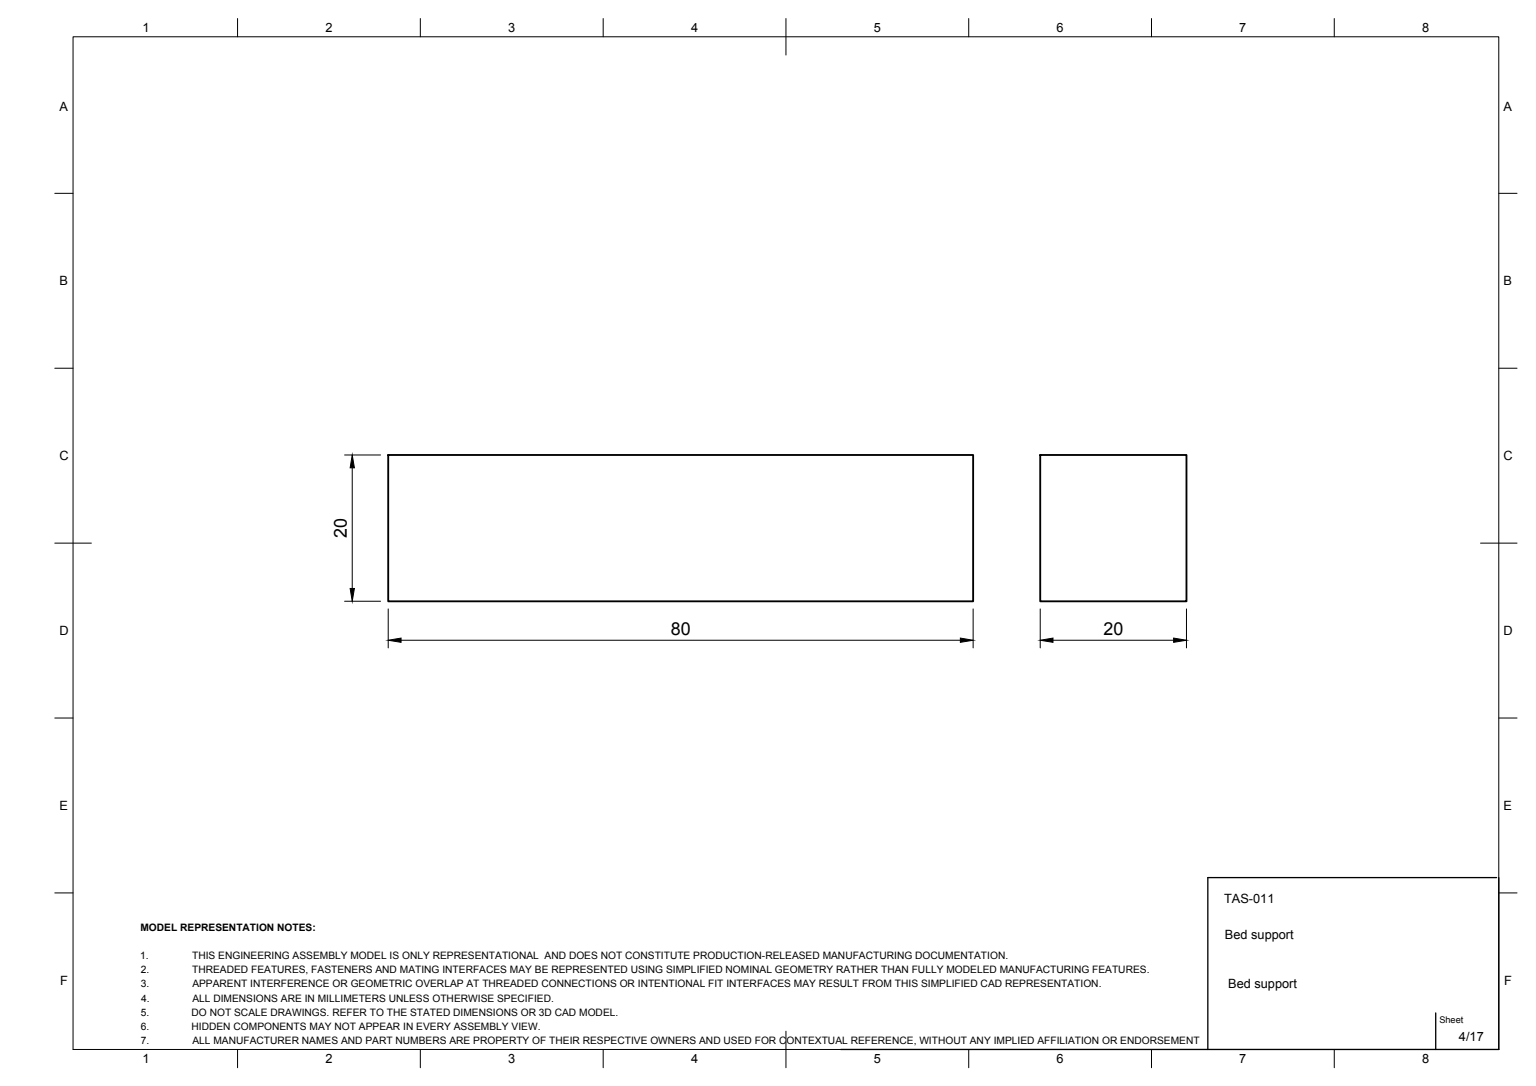
ISO-10303-21;
HEADER;
/* Generated by software containing ST-Developer
 * from STEP Tools, Inc. (www.steptools.com) 
 */

FILE_DESCRIPTION(
/* description */ (
'Independent manual bench leaf bending machine,200mm work width. Fabri
cated welded frame and folding leaf, repeated bushed and fully retaine
d hinge hardware, two handles with bonded grips, beveled clamping beam
 and modeledM12 clamp screws.2mm omitted-workpiece assembly reference 
gap, not a capacity claim. Native135deg hinge travel. Weld sizing, pro
duction fits, material condition, bending capacity, strength and life 
unassigned.'),
/* implementation_level */ '2;1');

FILE_NAME(
/* name */ 'Bed support.step',
/* time_stamp */ '2026-11-14T09:11:34-08:00',
/* author */ (''),
/* organization */ (''),
/* preprocessor_version */ 'ST-DEVELOPER v20.2',
/* originating_system */ 'Autodesk Translation Framework v15.17.0.0',
/* authorisation */ '');

FILE_SCHEMA (('AUTOMOTIVE_DESIGN { 1 0 10303 214 3 1 1 }'));
ENDSEC;

DATA;
#10=MECHANICAL_DESIGN_GEOMETRIC_PRESENTATION_REPRESENTATION('',(#450),#37701);
#414=SHAPE_REPRESENTATION_RELATIONSHIP('SRR','None',#37783,#432);
#432=ADVANCED_BREP_SHAPE_REPRESENTATION('',(#468),#37687);
#450=STYLED_ITEM('',(#37882),#468);
#468=MANIFOLD_SOLID_BREP('Body1',#4148);
#540=PLANE('',#4435);
#541=PLANE('',#4436);
#542=PLANE('',#4437);
#543=PLANE('',#4438);
#544=PLANE('',#4439);
#545=PLANE('',#4440);
#642=FACE_OUTER_BOUND('',#870,.T.);
#643=FACE_OUTER_BOUND('',#871,.T.);
#644=FACE_OUTER_BOUND('',#872,.T.);
#645=FACE_OUTER_BOUND('',#873,.T.);
#646=FACE_OUTER_BOUND('',#874,.T.);
#647=FACE_OUTER_BOUND('',#875,.T.);
#870=EDGE_LOOP('',(#2823,#2824,#2825,#2826));
#871=EDGE_LOOP('',(#2827,#2828,#2829,#2830));
#872=EDGE_LOOP('',(#2831,#2832,#2833,#2834));
#873=EDGE_LOOP('',(#2835,#2836,#2837,#2838));
#874=EDGE_LOOP('',(#2839,#2840,#2841,#2842));
#875=EDGE_LOOP('',(#2843,#2844,#2845,#2846));
#1124=LINE('',#5849,#1373);
#1125=LINE('',#5851,#1374);
#1126=LINE('',#5853,#1375);
#1127=LINE('',#5854,#1376);
#1128=LINE('',#5857,#1377);
#1129=LINE('',#5859,#1378);
#1130=LINE('',#5860,#1379);
#1131=LINE('',#5863,#1380);
#1132=LINE('',#5865,#1381);
#1133=LINE('',#5866,#1382);
#1134=LINE('',#5868,#1383);
#1135=LINE('',#5869,#1384);
#1373=VECTOR('',#4921,10.);
#1374=VECTOR('',#4922,10.);
#1375=VECTOR('',#4923,10.);
#1376=VECTOR('',#4924,10.);
#1377=VECTOR('',#4927,10.);
#1378=VECTOR('',#4928,10.);
#1379=VECTOR('',#4929,10.);
#1380=VECTOR('',#4932,10.);
#1381=VECTOR('',#4933,10.);
#1382=VECTOR('',#4934,10.);
#1383=VECTOR('',#4937,10.);
#1384=VECTOR('',#4938,10.);
#1697=VERTEX_POINT('',#5847);
#1698=VERTEX_POINT('',#5848);
#1699=VERTEX_POINT('',#5850);
#1700=VERTEX_POINT('',#5852);
#1701=VERTEX_POINT('',#5856);
#1702=VERTEX_POINT('',#5858);
#1703=VERTEX_POINT('',#5862);
#1704=VERTEX_POINT('',#5864);
#2145=EDGE_CURVE('',#1697,#1698,#1124,.T.);
#2146=EDGE_CURVE('',#1698,#1699,#1125,.T.);
#2147=EDGE_CURVE('',#1700,#1699,#1126,.T.);
#2148=EDGE_CURVE('',#1697,#1700,#1127,.T.);
#2149=EDGE_CURVE('',#1701,#1697,#1128,.T.);
#2150=EDGE_CURVE('',#1702,#1700,#1129,.T.);
#2151=EDGE_CURVE('',#1701,#1702,#1130,.T.);
#2152=EDGE_CURVE('',#1703,#1701,#1131,.T.);
#2153=EDGE_CURVE('',#1704,#1702,#1132,.T.);
#2154=EDGE_CURVE('',#1703,#1704,#1133,.T.);
#2155=EDGE_CURVE('',#1698,#1703,#1134,.T.);
#2156=EDGE_CURVE('',#1699,#1704,#1135,.T.);
#2823=ORIENTED_EDGE('',*,*,#2145,.T.);
#2824=ORIENTED_EDGE('',*,*,#2146,.T.);
#2825=ORIENTED_EDGE('',*,*,#2147,.F.);
#2826=ORIENTED_EDGE('',*,*,#2148,.F.);
#2827=ORIENTED_EDGE('',*,*,#2149,.T.);
#2828=ORIENTED_EDGE('',*,*,#2148,.T.);
#2829=ORIENTED_EDGE('',*,*,#2150,.F.);
#2830=ORIENTED_EDGE('',*,*,#2151,.F.);
#2831=ORIENTED_EDGE('',*,*,#2152,.T.);
#2832=ORIENTED_EDGE('',*,*,#2151,.T.);
#2833=ORIENTED_EDGE('',*,*,#2153,.F.);
#2834=ORIENTED_EDGE('',*,*,#2154,.F.);
#2835=ORIENTED_EDGE('',*,*,#2155,.T.);
#2836=ORIENTED_EDGE('',*,*,#2154,.T.);
#2837=ORIENTED_EDGE('',*,*,#2156,.F.);
#2838=ORIENTED_EDGE('',*,*,#2146,.F.);
#2839=ORIENTED_EDGE('',*,*,#2156,.T.);
#2840=ORIENTED_EDGE('',*,*,#2153,.T.);
#2841=ORIENTED_EDGE('',*,*,#2150,.T.);
#2842=ORIENTED_EDGE('',*,*,#2147,.T.);
#2843=ORIENTED_EDGE('',*,*,#2155,.F.);
#2844=ORIENTED_EDGE('',*,*,#2145,.F.);
#2845=ORIENTED_EDGE('',*,*,#2149,.F.);
#2846=ORIENTED_EDGE('',*,*,#2152,.F.);
#3972=ADVANCED_FACE('',(#642),#540,.T.);
#3973=ADVANCED_FACE('',(#643),#541,.T.);
#3974=ADVANCED_FACE('',(#644),#542,.T.);
#3975=ADVANCED_FACE('',(#645),#543,.T.);
#3976=ADVANCED_FACE('',(#646),#544,.T.);
#3977=ADVANCED_FACE('',(#647),#545,.F.);
#4148=CLOSED_SHELL('',(#3972,#3973,#3974,#3975,#3976,#3977));
#4434=AXIS2_PLACEMENT_3D('',#5845,#4917,#4918);
#4435=AXIS2_PLACEMENT_3D('',#5846,#4919,#4920);
#4436=AXIS2_PLACEMENT_3D('',#5855,#4925,#4926);
#4437=AXIS2_PLACEMENT_3D('',#5861,#4930,#4931);
#4438=AXIS2_PLACEMENT_3D('',#5867,#4935,#4936);
#4439=AXIS2_PLACEMENT_3D('',#5870,#4939,#4940);
#4440=AXIS2_PLACEMENT_3D('',#5871,#4941,#4942);
#4917=DIRECTION('axis',(0.,0.,1.));
#4918=DIRECTION('refdir',(1.,0.,0.));
#4919=DIRECTION('center_axis',(0.,1.,0.));
#4920=DIRECTION('ref_axis',(-1.,0.,0.));
#4921=DIRECTION('',(-1.,0.,0.));
#4922=DIRECTION('',(0.,0.,1.));
#4923=DIRECTION('',(-1.,0.,0.));
#4924=DIRECTION('',(0.,0.,1.));
#4925=DIRECTION('center_axis',(1.,0.,0.));
#4926=DIRECTION('ref_axis',(0.,1.,0.));
#4927=DIRECTION('',(0.,1.,0.));
#4928=DIRECTION('',(0.,1.,0.));
#4929=DIRECTION('',(0.,0.,1.));
#4930=DIRECTION('center_axis',(0.,-1.,0.));
#4931=DIRECTION('ref_axis',(1.,0.,0.));
#4932=DIRECTION('',(1.,0.,0.));
#4933=DIRECTION('',(1.,0.,0.));
#4934=DIRECTION('',(0.,0.,1.));
#4935=DIRECTION('center_axis',(-1.,0.,0.));
#4936=DIRECTION('ref_axis',(0.,-1.,0.));
#4937=DIRECTION('',(0.,-1.,0.));
#4938=DIRECTION('',(0.,-1.,0.));
#4939=DIRECTION('center_axis',(0.,0.,1.));
#4940=DIRECTION('ref_axis',(1.,0.,0.));
#4941=DIRECTION('center_axis',(0.,0.,1.));
#4942=DIRECTION('ref_axis',(1.,0.,0.));
#5845=CARTESIAN_POINT('',(0.,0.,0.));
#5846=CARTESIAN_POINT('Origin',(-10.,10.,10.));
#5847=CARTESIAN_POINT('',(-10.,10.,10.));
#5848=CARTESIAN_POINT('',(-90.,10.,10.));
#5849=CARTESIAN_POINT('',(-10.,10.,10.));
#5850=CARTESIAN_POINT('',(-90.,10.,30.));
#5851=CARTESIAN_POINT('',(-90.,10.,10.));
#5852=CARTESIAN_POINT('',(-10.,10.,30.));
#5853=CARTESIAN_POINT('',(-10.,10.,30.));
#5854=CARTESIAN_POINT('',(-10.,10.,10.));
#5855=CARTESIAN_POINT('Origin',(-10.,-10.,10.));
#5856=CARTESIAN_POINT('',(-10.,-10.,10.));
#5857=CARTESIAN_POINT('',(-10.,-10.,10.));
#5858=CARTESIAN_POINT('',(-10.,-10.,30.));
#5859=CARTESIAN_POINT('',(-10.,-10.,30.));
#5860=CARTESIAN_POINT('',(-10.,-10.,10.));
#5861=CARTESIAN_POINT('Origin',(-90.,-10.,10.));
#5862=CARTESIAN_POINT('',(-90.,-10.,10.));
#5863=CARTESIAN_POINT('',(-90.,-10.,10.));
#5864=CARTESIAN_POINT('',(-90.,-10.,30.));
#5865=CARTESIAN_POINT('',(-90.,-10.,30.));
#5866=CARTESIAN_POINT('',(-90.,-10.,10.));
#5867=CARTESIAN_POINT('Origin',(-90.,10.,10.));
#5868=CARTESIAN_POINT('',(-90.,10.,10.));
#5869=CARTESIAN_POINT('',(-90.,10.,30.));
#5870=CARTESIAN_POINT('Origin',(-50.,0.,30.));
#5871=CARTESIAN_POINT('Origin',(-50.,0.,10.));
#37667=UNCERTAINTY_MEASURE_WITH_UNIT(LENGTH_MEASURE(0.01),#37702,
'DISTANCE_ACCURACY_VALUE',
'Maximum model space distance between geometric entities at asserted c
onnectivities');
#37681=UNCERTAINTY_MEASURE_WITH_UNIT(LENGTH_MEASURE(0.01),#37702,
'DISTANCE_ACCURACY_VALUE',
'Maximum model space distance between geometric entities at asserted c
onnectivities');
#37687=(
GEOMETRIC_REPRESENTATION_CONTEXT(3)
GLOBAL_UNCERTAINTY_ASSIGNED_CONTEXT((#37667))
GLOBAL_UNIT_ASSIGNED_CONTEXT((#37702,#37704,#37705))
REPRESENTATION_CONTEXT('','3D')
);
#37701=(
GEOMETRIC_REPRESENTATION_CONTEXT(3)
GLOBAL_UNCERTAINTY_ASSIGNED_CONTEXT((#37681))
GLOBAL_UNIT_ASSIGNED_CONTEXT((#37702,#37704,#37705))
REPRESENTATION_CONTEXT('','3D')
);
#37702=(
LENGTH_UNIT()
NAMED_UNIT(*)
SI_UNIT(.MILLI.,.METRE.)
);
#37704=(
NAMED_UNIT(*)
PLANE_ANGLE_UNIT()
SI_UNIT($,.RADIAN.)
);
#37705=(
NAMED_UNIT(*)
SI_UNIT($,.STERADIAN.)
SOLID_ANGLE_UNIT()
);
#37711=SHAPE_DEFINITION_REPRESENTATION(#37730,#37783);
#37730=PRODUCT_DEFINITION_SHAPE('',$,#37803);
#37783=SHAPE_REPRESENTATION('',(#4434),#37687);
#37797=PRODUCT_DEFINITION_CONTEXT('part definition',#37856,'design');
#37803=PRODUCT_DEFINITION('Bed support','Bed support',#37822,#37797);
#37822=PRODUCT_DEFINITION_FORMATION('',$,#37863);
#37856=APPLICATION_CONTEXT(
'Core Data for Automotive Mechanical Design Process');
#37857=PRODUCT_CONTEXT('part definition',#37856,'mechanical');
#37863=PRODUCT('Bed support','Bed support',$,(#37857));
#37882=PRESENTATION_STYLE_ASSIGNMENT((#37890));
#37890=SURFACE_STYLE_USAGE(.BOTH.,#37898);
#37898=SURFACE_SIDE_STYLE('',(#37906));
#37906=SURFACE_STYLE_FILL_AREA(#37914);
#37914=FILL_AREA_STYLE('Opaque(169,212,242)',(#37922));
#37922=FILL_AREA_STYLE_COLOUR('Opaque(169,212,242)',#37930);
#37930=COLOUR_RGB('Opaque(169,212,242)',0.662745098039216,0.831372549019608,
0.949019607843137);
ENDSEC;
END-ISO-10303-21;
